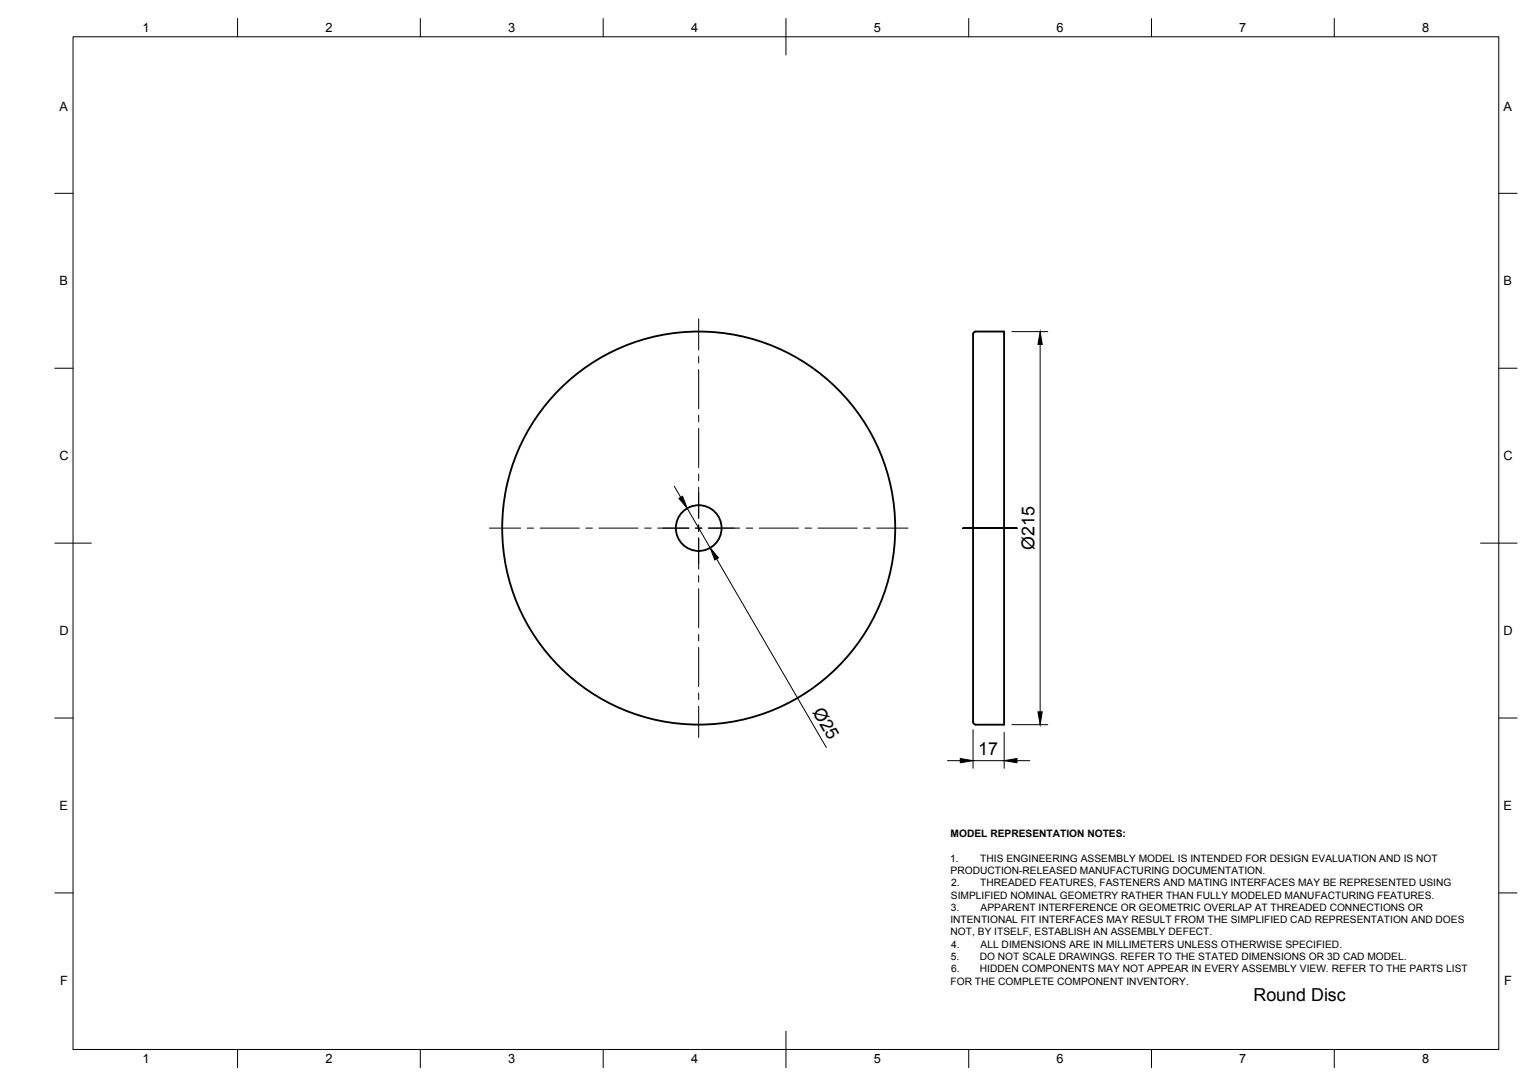
ISO-10303-21;
HEADER;
/* Generated by software containing ST-Developer
 * from STEP Tools, Inc. (www.steptools.com) 
 */

FILE_DESCRIPTION(
/* description */ ('STEP AP214'),
/* implementation_level */ '2;1');

FILE_NAME(
/* name */ 'ROUND DISC.step',
/* time_stamp */ '2026-10-06T11:20:11-07:00',
/* author */ (''),
/* organization */ (''),
/* preprocessor_version */ 'ST-DEVELOPER v20.2',
/* originating_system */ 'Autodesk Translation Framework v15.15.0.0',
/* authorisation */ '');

FILE_SCHEMA (('AUTOMOTIVE_DESIGN { 1 0 10303 214 3 1 1 }'));
ENDSEC;

DATA;
#10=MECHANICAL_DESIGN_GEOMETRIC_PRESENTATION_REPRESENTATION('',(#48),#2840);
#36=SHAPE_REPRESENTATION_RELATIONSHIP('SRR','None',#2867,#42);
#42=ADVANCED_BREP_SHAPE_REPRESENTATION('',(#54),#2835);
#48=STYLED_ITEM('',(#2905),#54);
#54=MANIFOLD_SOLID_BREP('Body1',#1548);
#67=TOROIDAL_SURFACE('',#1700,106.,1.5);
#79=FACE_BOUND('',#261,.T.);
#80=FACE_BOUND('',#263,.T.);
#105=PLANE('',#1707);
#106=PLANE('',#1708);
#158=FACE_OUTER_BOUND('',#257,.T.);
#159=FACE_OUTER_BOUND('',#258,.T.);
#160=FACE_OUTER_BOUND('',#259,.T.);
#161=FACE_OUTER_BOUND('',#260,.T.);
#162=FACE_OUTER_BOUND('',#262,.T.);
#257=EDGE_LOOP('',(#1126,#1127,#1128,#1129));
#258=EDGE_LOOP('',(#1130,#1131,#1132,#1133,#1134));
#259=EDGE_LOOP('',(#1135,#1136,#1137,#1138,#1139));
#260=EDGE_LOOP('',(#1140));
#261=EDGE_LOOP('',(#1141));
#262=EDGE_LOOP('',(#1142));
#263=EDGE_LOOP('',(#1143));
#363=LINE('',#2528,#456);
#364=LINE('',#2541,#457);
#456=VECTOR('',#2028,12.5);
#457=VECTOR('',#2045,107.5);
#562=CIRCLE('',#1698,12.5);
#563=CIRCLE('',#1699,12.5);
#564=CIRCLE('',#1701,106.);
#565=CIRCLE('',#1702,1.5);
#566=CIRCLE('',#1703,107.5);
#567=CIRCLE('',#1704,107.5);
#568=CIRCLE('',#1706,107.5);
#680=VERTEX_POINT('',#2525);
#681=VERTEX_POINT('',#2527);
#682=VERTEX_POINT('',#2531);
#683=VERTEX_POINT('',#2533);
#684=VERTEX_POINT('',#2535);
#685=VERTEX_POINT('',#2539);
#844=EDGE_CURVE('',#680,#680,#562,.T.);
#845=EDGE_CURVE('',#680,#681,#363,.T.);
#846=EDGE_CURVE('',#681,#681,#563,.T.);
#847=EDGE_CURVE('',#682,#682,#564,.T.);
#848=EDGE_CURVE('',#682,#683,#565,.T.);
#849=EDGE_CURVE('',#684,#683,#566,.T.);
#850=EDGE_CURVE('',#683,#684,#567,.T.);
#851=EDGE_CURVE('',#685,#685,#568,.T.);
#852=EDGE_CURVE('',#685,#684,#364,.T.);
#1126=ORIENTED_EDGE('',*,*,#844,.F.);
#1127=ORIENTED_EDGE('',*,*,#845,.T.);
#1128=ORIENTED_EDGE('',*,*,#846,.T.);
#1129=ORIENTED_EDGE('',*,*,#845,.F.);
#1130=ORIENTED_EDGE('',*,*,#847,.F.);
#1131=ORIENTED_EDGE('',*,*,#848,.T.);
#1132=ORIENTED_EDGE('',*,*,#849,.F.);
#1133=ORIENTED_EDGE('',*,*,#850,.F.);
#1134=ORIENTED_EDGE('',*,*,#848,.F.);
#1135=ORIENTED_EDGE('',*,*,#851,.T.);
#1136=ORIENTED_EDGE('',*,*,#852,.T.);
#1137=ORIENTED_EDGE('',*,*,#849,.T.);
#1138=ORIENTED_EDGE('',*,*,#850,.T.);
#1139=ORIENTED_EDGE('',*,*,#852,.F.);
#1140=ORIENTED_EDGE('',*,*,#847,.T.);
#1141=ORIENTED_EDGE('',*,*,#846,.F.);
#1142=ORIENTED_EDGE('',*,*,#851,.F.);
#1143=ORIENTED_EDGE('',*,*,#844,.T.);
#1423=CYLINDRICAL_SURFACE('',#1697,12.5);
#1424=CYLINDRICAL_SURFACE('',#1705,107.5);
#1489=ADVANCED_FACE('',(#158),#1423,.F.);
#1490=ADVANCED_FACE('',(#159),#67,.T.);
#1491=ADVANCED_FACE('',(#160),#1424,.T.);
#1492=ADVANCED_FACE('',(#161,#79),#105,.T.);
#1493=ADVANCED_FACE('',(#162,#80),#106,.F.);
#1548=CLOSED_SHELL('',(#1489,#1490,#1491,#1492,#1493));
#1696=AXIS2_PLACEMENT_3D('',#2523,#2022,#2023);
#1697=AXIS2_PLACEMENT_3D('',#2524,#2024,#2025);
#1698=AXIS2_PLACEMENT_3D('',#2526,#2026,#2027);
#1699=AXIS2_PLACEMENT_3D('',#2529,#2029,#2030);
#1700=AXIS2_PLACEMENT_3D('',#2530,#2031,#2032);
#1701=AXIS2_PLACEMENT_3D('',#2532,#2033,#2034);
#1702=AXIS2_PLACEMENT_3D('',#2534,#2035,#2036);
#1703=AXIS2_PLACEMENT_3D('',#2536,#2037,#2038);
#1704=AXIS2_PLACEMENT_3D('',#2537,#2039,#2040);
#1705=AXIS2_PLACEMENT_3D('',#2538,#2041,#2042);
#1706=AXIS2_PLACEMENT_3D('',#2540,#2043,#2044);
#1707=AXIS2_PLACEMENT_3D('',#2542,#2046,#2047);
#1708=AXIS2_PLACEMENT_3D('',#2543,#2048,#2049);
#2022=DIRECTION('axis',(0.,0.,1.));
#2023=DIRECTION('refdir',(1.,0.,0.));
#2024=DIRECTION('center_axis',(0.,1.,0.));
#2025=DIRECTION('ref_axis',(0.,0.,1.));
#2026=DIRECTION('center_axis',(0.,1.,0.));
#2027=DIRECTION('ref_axis',(0.,0.,1.));
#2028=DIRECTION('',(0.,1.,0.));
#2029=DIRECTION('center_axis',(0.,1.,0.));
#2030=DIRECTION('ref_axis',(0.,0.,1.));
#2031=DIRECTION('center_axis',(0.,1.,0.));
#2032=DIRECTION('ref_axis',(0.,0.,1.));
#2033=DIRECTION('center_axis',(0.,1.,0.));
#2034=DIRECTION('ref_axis',(0.,0.,1.));
#2035=DIRECTION('center_axis',(-1.,0.,0.));
#2036=DIRECTION('ref_axis',(0.,0.,-1.));
#2037=DIRECTION('center_axis',(0.,-1.,0.));
#2038=DIRECTION('ref_axis',(0.,0.,1.));
#2039=DIRECTION('center_axis',(0.,-1.,0.));
#2040=DIRECTION('ref_axis',(0.,0.,1.));
#2041=DIRECTION('center_axis',(0.,-1.,0.));
#2042=DIRECTION('ref_axis',(0.,0.,-1.));
#2043=DIRECTION('center_axis',(0.,1.,0.));
#2044=DIRECTION('ref_axis',(0.,0.,1.));
#2045=DIRECTION('',(0.,1.,0.));
#2046=DIRECTION('center_axis',(0.,1.,0.));
#2047=DIRECTION('ref_axis',(-1.38777878078145E-17,0.,1.));
#2048=DIRECTION('center_axis',(0.,1.,0.));
#2049=DIRECTION('ref_axis',(-1.38777878078145E-17,0.,1.));
#2523=CARTESIAN_POINT('',(0.,0.,0.));
#2524=CARTESIAN_POINT('Origin',(296.23500439103,-43.,-495.721631563692));
#2525=CARTESIAN_POINT('',(296.23500439103,0.,-508.221631563692));
#2526=CARTESIAN_POINT('Origin',(296.23500439103,0.,-495.721631563692));
#2527=CARTESIAN_POINT('',(296.23500439103,17.,-508.221631563692));
#2528=CARTESIAN_POINT('',(296.23500439103,-43.,-508.221631563692));
#2529=CARTESIAN_POINT('Origin',(296.23500439103,17.,-495.721631563692));
#2530=CARTESIAN_POINT('Origin',(296.235004391031,15.5,-495.721631563692));
#2531=CARTESIAN_POINT('',(296.235004391031,17.,-601.721631563692));
#2532=CARTESIAN_POINT('Origin',(296.235004391031,17.,-495.721631563692));
#2533=CARTESIAN_POINT('',(296.235004391031,15.5,-603.221631563692));
#2534=CARTESIAN_POINT('Origin',(296.235004391031,15.5,-601.721631563692));
#2535=CARTESIAN_POINT('',(296.235004391031,15.5,-388.221631563692));
#2536=CARTESIAN_POINT('Origin',(296.235004391031,15.5,-495.721631563692));
#2537=CARTESIAN_POINT('Origin',(296.235004391031,15.5,-495.721631563692));
#2538=CARTESIAN_POINT('Origin',(296.235004391031,17.,-495.721631563692));
#2539=CARTESIAN_POINT('',(296.235004391031,2.22044604925031E-15,-388.221631563692));
#2540=CARTESIAN_POINT('Origin',(296.235004391031,0.,-495.721631563692));
#2541=CARTESIAN_POINT('',(296.235004391031,17.,-388.221631563692));
#2542=CARTESIAN_POINT('Origin',(296.235004391031,17.,-495.721631563692));
#2543=CARTESIAN_POINT('Origin',(296.235004391031,0.,-495.721631563692));
#2827=UNCERTAINTY_MEASURE_WITH_UNIT(LENGTH_MEASURE(0.01),#2841,
'DISTANCE_ACCURACY_VALUE',
'Maximum model space distance between geometric entities at asserted c
onnectivities');
#2832=UNCERTAINTY_MEASURE_WITH_UNIT(LENGTH_MEASURE(0.01),#2841,
'DISTANCE_ACCURACY_VALUE',
'Maximum model space distance between geometric entities at asserted c
onnectivities');
#2835=(
GEOMETRIC_REPRESENTATION_CONTEXT(3)
GLOBAL_UNCERTAINTY_ASSIGNED_CONTEXT((#2827))
GLOBAL_UNIT_ASSIGNED_CONTEXT((#2841,#2843,#2844))
REPRESENTATION_CONTEXT('','3D')
);
#2840=(
GEOMETRIC_REPRESENTATION_CONTEXT(3)
GLOBAL_UNCERTAINTY_ASSIGNED_CONTEXT((#2832))
GLOBAL_UNIT_ASSIGNED_CONTEXT((#2841,#2843,#2844))
REPRESENTATION_CONTEXT('','3D')
);
#2841=(
LENGTH_UNIT()
NAMED_UNIT(*)
SI_UNIT(.MILLI.,.METRE.)
);
#2843=(
NAMED_UNIT(*)
PLANE_ANGLE_UNIT()
SI_UNIT($,.RADIAN.)
);
#2844=(
NAMED_UNIT(*)
SI_UNIT($,.STERADIAN.)
SOLID_ANGLE_UNIT()
);
#2847=SHAPE_DEFINITION_REPRESENTATION(#2854,#2867);
#2854=PRODUCT_DEFINITION_SHAPE('',$,#2875);
#2867=SHAPE_REPRESENTATION('',(#1696),#2835);
#2872=PRODUCT_DEFINITION_CONTEXT('part definition',#2895,'design');
#2875=PRODUCT_DEFINITION('ROUND DISC','ROUND DISC',#2882,#2872);
#2882=PRODUCT_DEFINITION_FORMATION('',$,#2899);
#2895=APPLICATION_CONTEXT(
'Core Data for Automotive Mechanical Design Process');
#2896=PRODUCT_CONTEXT('part definition',#2895,'mechanical');
#2899=PRODUCT('ROUND DISC','ROUND DISC',$,(#2896));
#2905=PRESENTATION_STYLE_ASSIGNMENT((#2907));
#2907=SURFACE_STYLE_USAGE(.BOTH.,#2909);
#2909=SURFACE_SIDE_STYLE('',(#2911));
#2911=SURFACE_STYLE_FILL_AREA(#2913);
#2913=FILL_AREA_STYLE('Opaque(202,209,238)',(#2915));
#2915=FILL_AREA_STYLE_COLOUR('Opaque(202,209,238)',#2917);
#2917=COLOUR_RGB('Opaque(202,209,238)', 0.66274510, 0.83137255, 0.94901961);
ENDSEC;
END-ISO-10303-21;
